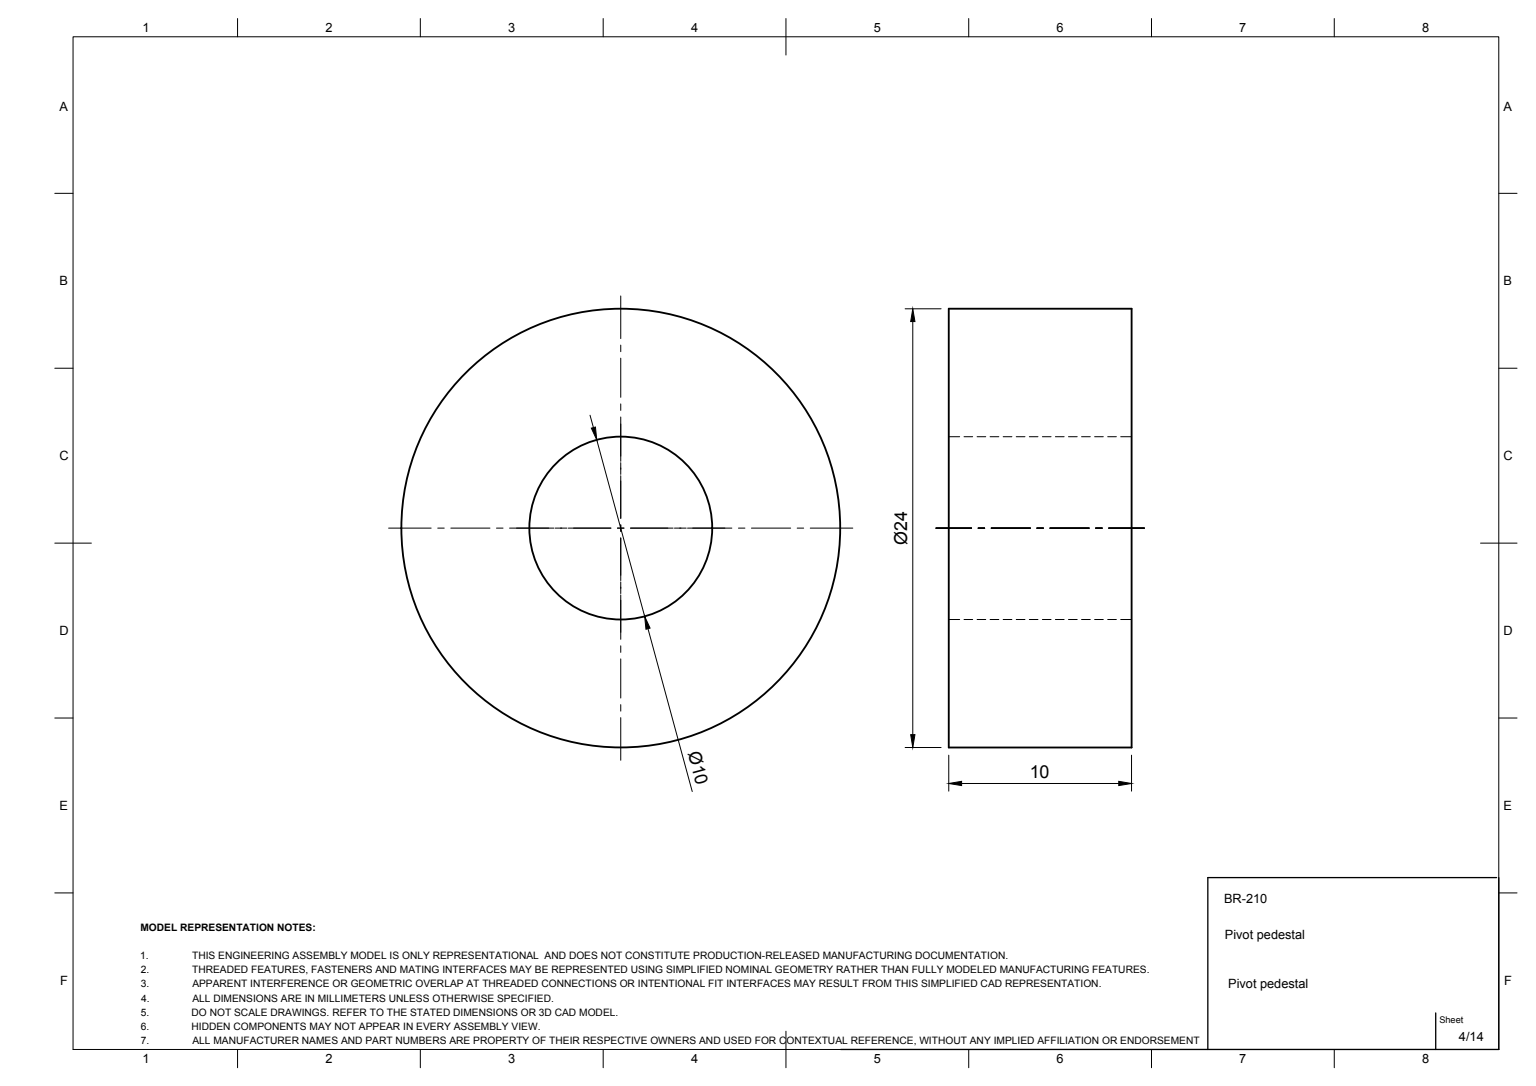
ISO-10303-21;
HEADER;
/* Generated by software containing ST-Developer
 * from STEP Tools, Inc. (www.steptools.com) 
 */

FILE_DESCRIPTION(
/* description */ ('Independent 1:2 reduction pantograph. 120 mm parallelogram sides; fix
ed fulcrum on the extension of a 240 mm link. Drawing point halfway al
ong its link, so its XY displacement is one half of the tracing point.
 Replaceable pivot bushes and retained pins. Calibration and productio
n accuracy unassigned.'),
/* implementation_level */ '2;1');

FILE_NAME(
/* name */ 'Pivot pedestal.step',
/* time_stamp */ '2026-11-07T22:11:57-08:00',
/* author */ (''),
/* organization */ (''),
/* preprocessor_version */ 'ST-DEVELOPER v20.2',
/* originating_system */ 'Autodesk Translation Framework v15.17.0.0',
/* authorisation */ '');

FILE_SCHEMA (('AUTOMOTIVE_DESIGN { 1 0 10303 214 3 1 1 }'));
ENDSEC;

DATA;
#10=MECHANICAL_DESIGN_GEOMETRIC_PRESENTATION_REPRESENTATION('',(#187),#2926);
#161=SHAPE_REPRESENTATION_RELATIONSHIP('SRR','None',#2998,#174);
#174=ADVANCED_BREP_SHAPE_REPRESENTATION('',(#200),#2914);
#187=STYLED_ITEM('',(#3072),#200);
#200=MANIFOLD_SOLID_BREP('Body1',#1542);
#222=FACE_BOUND('',#421,.T.);
#223=FACE_BOUND('',#423,.T.);
#264=PLANE('',#1728);
#265=PLANE('',#1729);
#316=FACE_OUTER_BOUND('',#418,.T.);
#317=FACE_OUTER_BOUND('',#419,.T.);
#318=FACE_OUTER_BOUND('',#420,.T.);
#319=FACE_OUTER_BOUND('',#422,.T.);
#418=EDGE_LOOP('',(#1121,#1122,#1123,#1124));
#419=EDGE_LOOP('',(#1125,#1126,#1127,#1128));
#420=EDGE_LOOP('',(#1129));
#421=EDGE_LOOP('',(#1130));
#422=EDGE_LOOP('',(#1131));
#423=EDGE_LOOP('',(#1132));
#552=LINE('',#2535,#633);
#553=LINE('',#2541,#634);
#633=VECTOR('',#1998,5.);
#634=VECTOR('',#2005,12.);
#707=CIRCLE('',#1723,5.);
#708=CIRCLE('',#1724,5.);
#709=CIRCLE('',#1726,12.);
#710=CIRCLE('',#1727,12.);
#803=VERTEX_POINT('',#2532);
#804=VERTEX_POINT('',#2534);
#805=VERTEX_POINT('',#2538);
#806=VERTEX_POINT('',#2540);
#925=EDGE_CURVE('',#803,#803,#707,.T.);
#926=EDGE_CURVE('',#803,#804,#552,.T.);
#927=EDGE_CURVE('',#804,#804,#708,.T.);
#928=EDGE_CURVE('',#805,#805,#709,.T.);
#929=EDGE_CURVE('',#805,#806,#553,.T.);
#930=EDGE_CURVE('',#806,#806,#710,.T.);
#1121=ORIENTED_EDGE('',*,*,#925,.F.);
#1122=ORIENTED_EDGE('',*,*,#926,.T.);
#1123=ORIENTED_EDGE('',*,*,#927,.T.);
#1124=ORIENTED_EDGE('',*,*,#926,.F.);
#1125=ORIENTED_EDGE('',*,*,#928,.F.);
#1126=ORIENTED_EDGE('',*,*,#929,.T.);
#1127=ORIENTED_EDGE('',*,*,#930,.T.);
#1128=ORIENTED_EDGE('',*,*,#929,.F.);
#1129=ORIENTED_EDGE('',*,*,#928,.T.);
#1130=ORIENTED_EDGE('',*,*,#925,.T.);
#1131=ORIENTED_EDGE('',*,*,#930,.F.);
#1132=ORIENTED_EDGE('',*,*,#927,.F.);
#1410=CYLINDRICAL_SURFACE('',#1722,5.);
#1411=CYLINDRICAL_SURFACE('',#1725,12.);
#1460=ADVANCED_FACE('',(#316),#1410,.F.);
#1461=ADVANCED_FACE('',(#317),#1411,.T.);
#1462=ADVANCED_FACE('',(#318,#222),#264,.T.);
#1463=ADVANCED_FACE('',(#319,#223),#265,.F.);
#1542=CLOSED_SHELL('',(#1460,#1461,#1462,#1463));
#1721=AXIS2_PLACEMENT_3D('',#2530,#1992,#1993);
#1722=AXIS2_PLACEMENT_3D('',#2531,#1994,#1995);
#1723=AXIS2_PLACEMENT_3D('',#2533,#1996,#1997);
#1724=AXIS2_PLACEMENT_3D('',#2536,#1999,#2000);
#1725=AXIS2_PLACEMENT_3D('',#2537,#2001,#2002);
#1726=AXIS2_PLACEMENT_3D('',#2539,#2003,#2004);
#1727=AXIS2_PLACEMENT_3D('',#2542,#2006,#2007);
#1728=AXIS2_PLACEMENT_3D('',#2543,#2008,#2009);
#1729=AXIS2_PLACEMENT_3D('',#2544,#2010,#2011);
#1992=DIRECTION('axis',(0.,0.,1.));
#1993=DIRECTION('refdir',(1.,0.,0.));
#1994=DIRECTION('center_axis',(0.,0.,1.));
#1995=DIRECTION('ref_axis',(1.,0.,0.));
#1996=DIRECTION('center_axis',(0.,0.,-1.));
#1997=DIRECTION('ref_axis',(1.,0.,0.));
#1998=DIRECTION('',(0.,0.,-1.));
#1999=DIRECTION('center_axis',(0.,0.,-1.));
#2000=DIRECTION('ref_axis',(1.,0.,0.));
#2001=DIRECTION('center_axis',(0.,0.,1.));
#2002=DIRECTION('ref_axis',(1.,0.,0.));
#2003=DIRECTION('center_axis',(0.,0.,1.));
#2004=DIRECTION('ref_axis',(1.,0.,0.));
#2005=DIRECTION('',(0.,0.,-1.));
#2006=DIRECTION('center_axis',(0.,0.,1.));
#2007=DIRECTION('ref_axis',(1.,0.,0.));
#2008=DIRECTION('center_axis',(0.,0.,1.));
#2009=DIRECTION('ref_axis',(1.,0.,0.));
#2010=DIRECTION('center_axis',(0.,0.,1.));
#2011=DIRECTION('ref_axis',(1.,0.,0.));
#2530=CARTESIAN_POINT('',(0.,0.,0.));
#2531=CARTESIAN_POINT('Origin',(0.,0.,0.));
#2532=CARTESIAN_POINT('',(-5.,-6.12323399573677E-16,10.));
#2533=CARTESIAN_POINT('Origin',(0.,0.,10.));
#2534=CARTESIAN_POINT('',(-5.,-6.12323399573677E-16,0.));
#2535=CARTESIAN_POINT('',(-5.,-6.12323399573677E-16,0.));
#2536=CARTESIAN_POINT('Origin',(0.,0.,0.));
#2537=CARTESIAN_POINT('Origin',(0.,0.,0.));
#2538=CARTESIAN_POINT('',(-12.,-1.46957615897682E-15,10.));
#2539=CARTESIAN_POINT('Origin',(0.,0.,10.));
#2540=CARTESIAN_POINT('',(-12.,-1.46957615897682E-15,0.));
#2541=CARTESIAN_POINT('',(-12.,-1.46957615897682E-15,0.));
#2542=CARTESIAN_POINT('Origin',(0.,0.,0.));
#2543=CARTESIAN_POINT('Origin',(0.,0.,10.));
#2544=CARTESIAN_POINT('Origin',(0.,0.,0.));
#2899=UNCERTAINTY_MEASURE_WITH_UNIT(LENGTH_MEASURE(0.01),#2927,
'DISTANCE_ACCURACY_VALUE',
'Maximum model space distance between geometric entities at asserted c
onnectivities');
#2911=UNCERTAINTY_MEASURE_WITH_UNIT(LENGTH_MEASURE(0.01),#2927,
'DISTANCE_ACCURACY_VALUE',
'Maximum model space distance between geometric entities at asserted c
onnectivities');
#2914=(
GEOMETRIC_REPRESENTATION_CONTEXT(3)
GLOBAL_UNCERTAINTY_ASSIGNED_CONTEXT((#2899))
GLOBAL_UNIT_ASSIGNED_CONTEXT((#2927,#2929,#2930))
REPRESENTATION_CONTEXT('','3D')
);
#2926=(
GEOMETRIC_REPRESENTATION_CONTEXT(3)
GLOBAL_UNCERTAINTY_ASSIGNED_CONTEXT((#2911))
GLOBAL_UNIT_ASSIGNED_CONTEXT((#2927,#2929,#2930))
REPRESENTATION_CONTEXT('','3D')
);
#2927=(
LENGTH_UNIT()
NAMED_UNIT(*)
SI_UNIT(.MILLI.,.METRE.)
);
#2929=(
NAMED_UNIT(*)
PLANE_ANGLE_UNIT()
SI_UNIT($,.RADIAN.)
);
#2930=(
NAMED_UNIT(*)
SI_UNIT($,.STERADIAN.)
SOLID_ANGLE_UNIT()
);
#2933=SHAPE_DEFINITION_REPRESENTATION(#2947,#2998);
#2947=PRODUCT_DEFINITION_SHAPE('',$,#3013);
#2998=SHAPE_REPRESENTATION('',(#1721),#2914);
#3010=PRODUCT_DEFINITION_CONTEXT('part definition',#3054,'design');
#3013=PRODUCT_DEFINITION('Pivot pedestal','Pivot pedestal',#3027,#3010);
#3027=PRODUCT_DEFINITION_FORMATION('',$,#3058);
#3054=APPLICATION_CONTEXT(
'Core Data for Automotive Mechanical Design Process');
#3055=PRODUCT_CONTEXT('part definition',#3054,'mechanical');
#3058=PRODUCT('Pivot pedestal','Pivot pedestal','Pivot pedestal',(#3055));
#3072=PRESENTATION_STYLE_ASSIGNMENT((#3084));
#3084=SURFACE_STYLE_USAGE(.BOTH.,#3096);
#3096=SURFACE_SIDE_STYLE('',(#3108));
#3108=SURFACE_STYLE_FILL_AREA(#3120);
#3120=FILL_AREA_STYLE('Pedestal gray',(#3132));
#3132=FILL_AREA_STYLE_COLOUR('Pedestal gray',#3144);
#3144=COLOUR_RGB('Pedestal gray',0.407843137254902,0.447058823529412,0.498039215686275);
ENDSEC;
END-ISO-10303-21;
